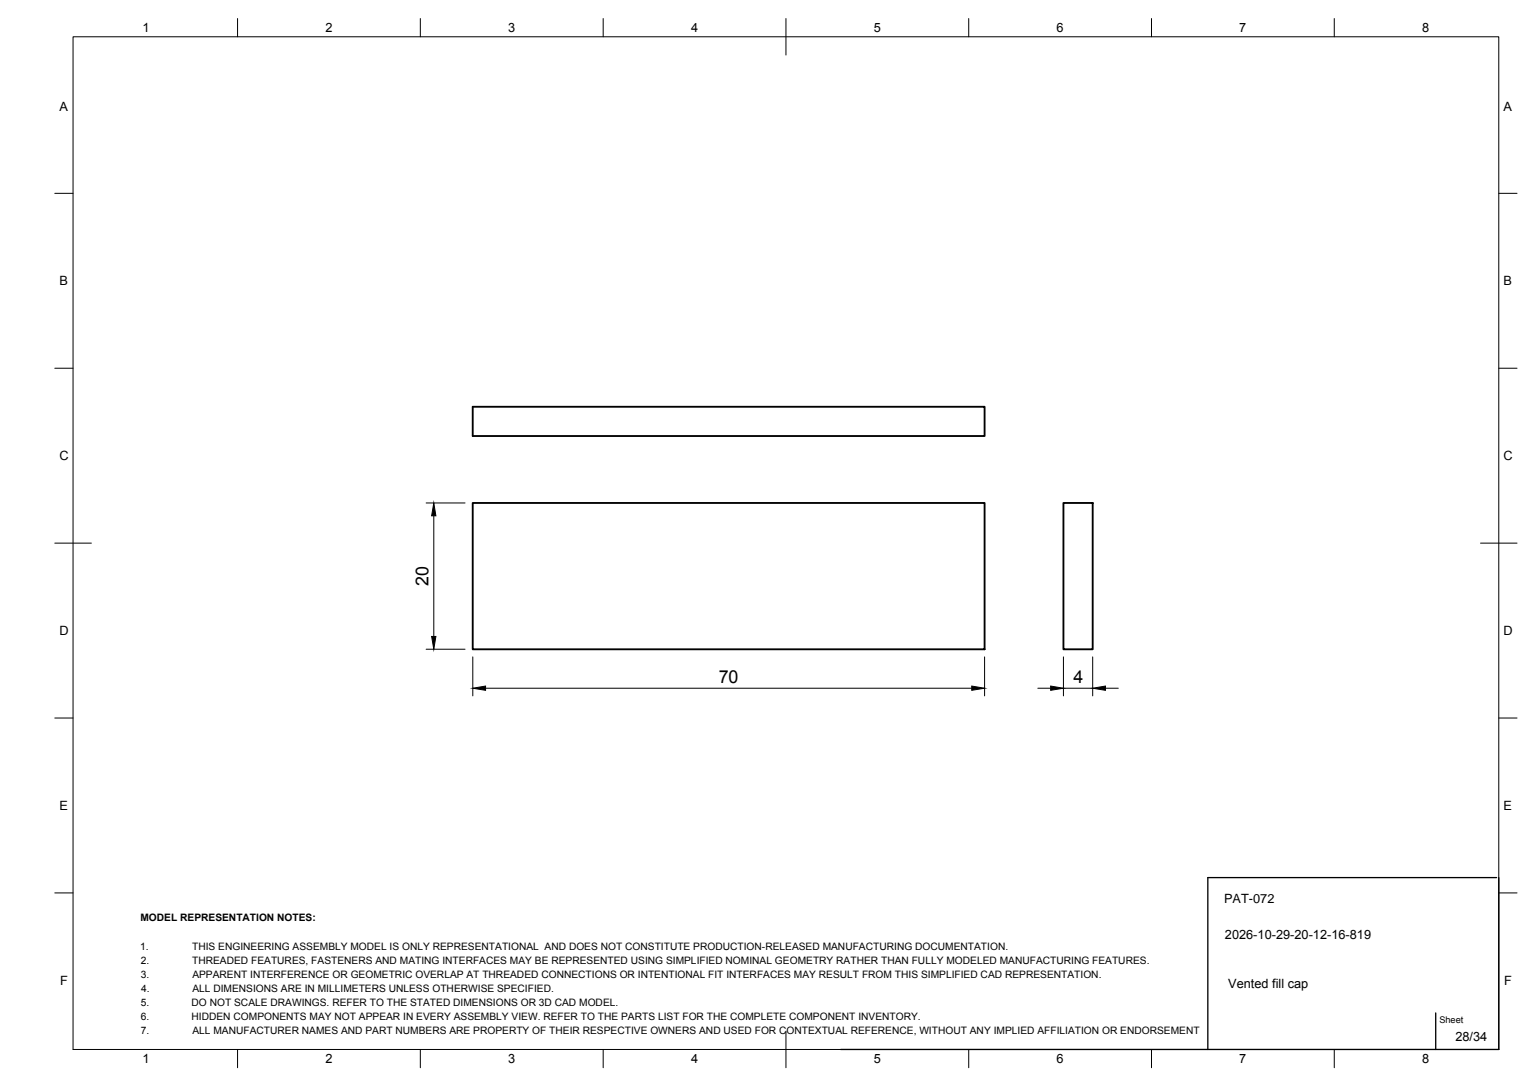
ISO-10303-21;
HEADER;
/* Generated by software containing ST-Developer
 * from STEP Tools, Inc. (www.steptools.com) 
 */

FILE_DESCRIPTION(
/* description */ ('PAT-072'),
/* implementation_level */ '2;1');

FILE_NAME(
/* name */ 'Vented fill cap.step',
/* time_stamp */ '2026-10-29T20:11:56-07:00',
/* author */ (''),
/* organization */ (''),
/* preprocessor_version */ 'ST-DEVELOPER v20.2',
/* originating_system */ 'Autodesk Translation Framework v15.17.0.0',
/* authorisation */ '');

FILE_SCHEMA (('AUTOMOTIVE_DESIGN { 1 0 10303 214 3 1 1 }'));
ENDSEC;

DATA;
#10=MECHANICAL_DESIGN_GEOMETRIC_PRESENTATION_REPRESENTATION('',(#360),#11432);
#288=SHAPE_REPRESENTATION_RELATIONSHIP('SRR','None',#11592,#324);
#324=ADVANCED_BREP_SHAPE_REPRESENTATION('',(#396),#11423);
#360=STYLED_ITEM('',(#11812),#396);
#396=MANIFOLD_SOLID_BREP('Body1',#6095);
#552=FACE_BOUND('',#1603,.T.);
#553=FACE_BOUND('',#1606,.T.);
#554=FACE_BOUND('',#1609,.T.);
#734=PLANE('',#7070);
#735=PLANE('',#7075);
#736=PLANE('',#7078);
#1079=FACE_OUTER_BOUND('',#1601,.T.);
#1080=FACE_OUTER_BOUND('',#1602,.T.);
#1081=FACE_OUTER_BOUND('',#1604,.T.);
#1082=FACE_OUTER_BOUND('',#1605,.T.);
#1083=FACE_OUTER_BOUND('',#1607,.T.);
#1084=FACE_OUTER_BOUND('',#1608,.T.);
#1601=EDGE_LOOP('',(#5222,#5223,#5224,#5225));
#1602=EDGE_LOOP('',(#5226));
#1603=EDGE_LOOP('',(#5227));
#1604=EDGE_LOOP('',(#5228,#5229,#5230,#5231));
#1605=EDGE_LOOP('',(#5232));
#1606=EDGE_LOOP('',(#5233));
#1607=EDGE_LOOP('',(#5234,#5235,#5236,#5237));
#1608=EDGE_LOOP('',(#5238));
#1609=EDGE_LOOP('',(#5239));
#2004=LINE('',#10935,#2423);
#2005=LINE('',#10945,#2424);
#2006=LINE('',#10949,#2425);
#2423=VECTOR('',#8689,0.075);
#2424=VECTOR('',#8702,1.);
#2425=VECTOR('',#8707,0.6);
#2791=CIRCLE('',#7068,0.075);
#2792=CIRCLE('',#7069,0.075);
#2793=CIRCLE('',#7071,1.);
#2794=CIRCLE('',#7072,0.6);
#2795=CIRCLE('',#7074,1.);
#2796=CIRCLE('',#7077,0.6);
#3214=VERTEX_POINT('',#10932);
#3215=VERTEX_POINT('',#10934);
#3216=VERTEX_POINT('',#10938);
#3217=VERTEX_POINT('',#10940);
#3218=VERTEX_POINT('',#10943);
#3219=VERTEX_POINT('',#10948);
#3900=EDGE_CURVE('',#3214,#3214,#2791,.T.);
#3901=EDGE_CURVE('',#3214,#3215,#2004,.T.);
#3902=EDGE_CURVE('',#3215,#3215,#2792,.T.);
#3903=EDGE_CURVE('',#3216,#3216,#2793,.T.);
#3904=EDGE_CURVE('',#3217,#3217,#2794,.T.);
#3905=EDGE_CURVE('',#3218,#3218,#2795,.T.);
#3906=EDGE_CURVE('',#3218,#3216,#2005,.T.);
#3907=EDGE_CURVE('',#3217,#3219,#2006,.T.);
#3908=EDGE_CURVE('',#3219,#3219,#2796,.T.);
#5222=ORIENTED_EDGE('',*,*,#3900,.F.);
#5223=ORIENTED_EDGE('',*,*,#3901,.T.);
#5224=ORIENTED_EDGE('',*,*,#3902,.F.);
#5225=ORIENTED_EDGE('',*,*,#3901,.F.);
#5226=ORIENTED_EDGE('',*,*,#3903,.F.);
#5227=ORIENTED_EDGE('',*,*,#3904,.T.);
#5228=ORIENTED_EDGE('',*,*,#3905,.F.);
#5229=ORIENTED_EDGE('',*,*,#3906,.T.);
#5230=ORIENTED_EDGE('',*,*,#3903,.T.);
#5231=ORIENTED_EDGE('',*,*,#3906,.F.);
#5232=ORIENTED_EDGE('',*,*,#3905,.T.);
#5233=ORIENTED_EDGE('',*,*,#3902,.T.);
#5234=ORIENTED_EDGE('',*,*,#3904,.F.);
#5235=ORIENTED_EDGE('',*,*,#3907,.T.);
#5236=ORIENTED_EDGE('',*,*,#3908,.T.);
#5237=ORIENTED_EDGE('',*,*,#3907,.F.);
#5238=ORIENTED_EDGE('',*,*,#3908,.F.);
#5239=ORIENTED_EDGE('',*,*,#3900,.T.);
#5677=CYLINDRICAL_SURFACE('',#7067,0.075);
#5678=CYLINDRICAL_SURFACE('',#7073,1.);
#5679=CYLINDRICAL_SURFACE('',#7076,0.6);
#5978=ADVANCED_FACE('',(#1079),#5677,.F.);
#5979=ADVANCED_FACE('',(#1080,#552),#734,.F.);
#5980=ADVANCED_FACE('',(#1081),#5678,.T.);
#5981=ADVANCED_FACE('',(#1082,#553),#735,.T.);
#5982=ADVANCED_FACE('',(#1083),#5679,.T.);
#5983=ADVANCED_FACE('',(#1084,#554),#736,.F.);
#6095=CLOSED_SHELL('',(#5978,#5979,#5980,#5981,#5982,#5983));
#7066=AXIS2_PLACEMENT_3D('',#10930,#8683,#8684);
#7067=AXIS2_PLACEMENT_3D('',#10931,#8685,#8686);
#7068=AXIS2_PLACEMENT_3D('',#10933,#8687,#8688);
#7069=AXIS2_PLACEMENT_3D('',#10936,#8690,#8691);
#7070=AXIS2_PLACEMENT_3D('',#10937,#8692,#8693);
#7071=AXIS2_PLACEMENT_3D('',#10939,#8694,#8695);
#7072=AXIS2_PLACEMENT_3D('',#10941,#8696,#8697);
#7073=AXIS2_PLACEMENT_3D('',#10942,#8698,#8699);
#7074=AXIS2_PLACEMENT_3D('',#10944,#8700,#8701);
#7075=AXIS2_PLACEMENT_3D('',#10946,#8703,#8704);
#7076=AXIS2_PLACEMENT_3D('',#10947,#8705,#8706);
#7077=AXIS2_PLACEMENT_3D('',#10950,#8708,#8709);
#7078=AXIS2_PLACEMENT_3D('',#10951,#8710,#8711);
#8683=DIRECTION('axis',(0.,0.,1.));
#8684=DIRECTION('refdir',(1.,0.,0.));
#8685=DIRECTION('center_axis',(0.,0.,1.));
#8686=DIRECTION('ref_axis',(1.,0.,0.));
#8687=DIRECTION('center_axis',(0.,0.,1.));
#8688=DIRECTION('ref_axis',(1.,0.,0.));
#8689=DIRECTION('',(0.,0.,1.));
#8690=DIRECTION('center_axis',(0.,0.,-1.));
#8691=DIRECTION('ref_axis',(1.,0.,0.));
#8692=DIRECTION('center_axis',(0.,0.,1.));
#8693=DIRECTION('ref_axis',(1.,0.,0.));
#8694=DIRECTION('center_axis',(0.,0.,1.));
#8695=DIRECTION('ref_axis',(1.,0.,0.));
#8696=DIRECTION('center_axis',(0.,0.,1.));
#8697=DIRECTION('ref_axis',(1.,0.,0.));
#8698=DIRECTION('center_axis',(0.,0.,1.));
#8699=DIRECTION('ref_axis',(1.,0.,0.));
#8700=DIRECTION('center_axis',(0.,0.,1.));
#8701=DIRECTION('ref_axis',(1.,0.,0.));
#8702=DIRECTION('',(0.,0.,-1.));
#8703=DIRECTION('center_axis',(0.,0.,1.));
#8704=DIRECTION('ref_axis',(1.,0.,0.));
#8705=DIRECTION('center_axis',(0.,0.,1.));
#8706=DIRECTION('ref_axis',(1.,0.,0.));
#8707=DIRECTION('',(0.,0.,-1.));
#8708=DIRECTION('center_axis',(0.,0.,1.));
#8709=DIRECTION('ref_axis',(1.,0.,0.));
#8710=DIRECTION('center_axis',(0.,0.,1.));
#8711=DIRECTION('ref_axis',(1.,0.,0.));
#10930=CARTESIAN_POINT('',(0.,0.,0.));
#10931=CARTESIAN_POINT('Origin',(0.,0.,15.1));
#10932=CARTESIAN_POINT('',(-0.075,-9.18485099360515E-18,15.2));
#10933=CARTESIAN_POINT('Origin',(0.,0.,15.2));
#10934=CARTESIAN_POINT('',(-0.075,9.18485099360515E-18,16.2));
#10935=CARTESIAN_POINT('',(-0.075,-9.18485099360515E-18,15.1));
#10936=CARTESIAN_POINT('Origin',(0.,0.,16.2));
#10937=CARTESIAN_POINT('Origin',(0.,0.,15.7));
#10938=CARTESIAN_POINT('',(-1.,-1.22464679914735E-16,15.7));
#10939=CARTESIAN_POINT('Origin',(0.,0.,15.7));
#10940=CARTESIAN_POINT('',(-0.6,-7.34788079488412E-17,15.7));
#10941=CARTESIAN_POINT('Origin',(0.,0.,15.7));
#10942=CARTESIAN_POINT('Origin',(0.,0.,15.7));
#10943=CARTESIAN_POINT('',(-1.,-1.22464679914735E-16,16.2));
#10944=CARTESIAN_POINT('Origin',(0.,0.,16.2));
#10945=CARTESIAN_POINT('',(-1.,-1.22464679914735E-16,15.7));
#10946=CARTESIAN_POINT('Origin',(0.,0.,16.2));
#10947=CARTESIAN_POINT('Origin',(0.,0.,15.2));
#10948=CARTESIAN_POINT('',(-0.6,-7.34788079488412E-17,15.2));
#10949=CARTESIAN_POINT('',(-0.6,-7.34788079488412E-17,15.2));
#10950=CARTESIAN_POINT('Origin',(0.,0.,15.2));
#10951=CARTESIAN_POINT('Origin',(0.,0.,15.2));
#11384=UNCERTAINTY_MEASURE_WITH_UNIT(LENGTH_MEASURE(0.001),#11433,
'DISTANCE_ACCURACY_VALUE',
'Maximum model space distance between geometric entities at asserted c
onnectivities');
#11393=UNCERTAINTY_MEASURE_WITH_UNIT(LENGTH_MEASURE(0.001),#11433,
'DISTANCE_ACCURACY_VALUE',
'Maximum model space distance between geometric entities at asserted c
onnectivities');
#11423=(
GEOMETRIC_REPRESENTATION_CONTEXT(3)
GLOBAL_UNCERTAINTY_ASSIGNED_CONTEXT((#11384))
GLOBAL_UNIT_ASSIGNED_CONTEXT((#11433,#11435,#11436))
REPRESENTATION_CONTEXT('','3D')
);
#11432=(
GEOMETRIC_REPRESENTATION_CONTEXT(3)
GLOBAL_UNCERTAINTY_ASSIGNED_CONTEXT((#11393))
GLOBAL_UNIT_ASSIGNED_CONTEXT((#11433,#11435,#11436))
REPRESENTATION_CONTEXT('','3D')
);
#11433=(
LENGTH_UNIT()
NAMED_UNIT(*)
SI_UNIT(.CENTI.,.METRE.)
);
#11435=(
NAMED_UNIT(*)
PLANE_ANGLE_UNIT()
SI_UNIT($,.RADIAN.)
);
#11436=(
NAMED_UNIT(*)
SI_UNIT($,.STERADIAN.)
SOLID_ANGLE_UNIT()
);
#11466=SHAPE_DEFINITION_REPRESENTATION(#11504,#11592);
#11504=PRODUCT_DEFINITION_SHAPE('',$,#11631);
#11592=SHAPE_REPRESENTATION('',(#7066),#11423);
#11601=PRODUCT_DEFINITION_CONTEXT('part definition',#11717,'design');
#11631=PRODUCT_DEFINITION('Vented fill cap','Vented fill cap',#11669,
#11601);
#11669=PRODUCT_DEFINITION_FORMATION('',$,#11748);
#11717=APPLICATION_CONTEXT(
'Core Data for Automotive Mechanical Design Process');
#11718=PRODUCT_CONTEXT('part definition',#11717,'mechanical');
#11748=PRODUCT('Vented fill cap','Vented fill cap',
'Vented fill cap',(#11718));
#11806=COLOUR_RGB('Sky Blue',0.24,0.69,0.87);
#11807=FILL_AREA_STYLE_COLOUR('',#11806);
#11808=FILL_AREA_STYLE('',(#11807));
#11809=SURFACE_STYLE_FILL_AREA(#11808);
#11810=SURFACE_SIDE_STYLE('',(#11809));
#11811=SURFACE_STYLE_USAGE(.BOTH.,#11810);
#11812=PRESENTATION_STYLE_ASSIGNMENT((#11811));
ENDSEC;
END-ISO-10303-21;
